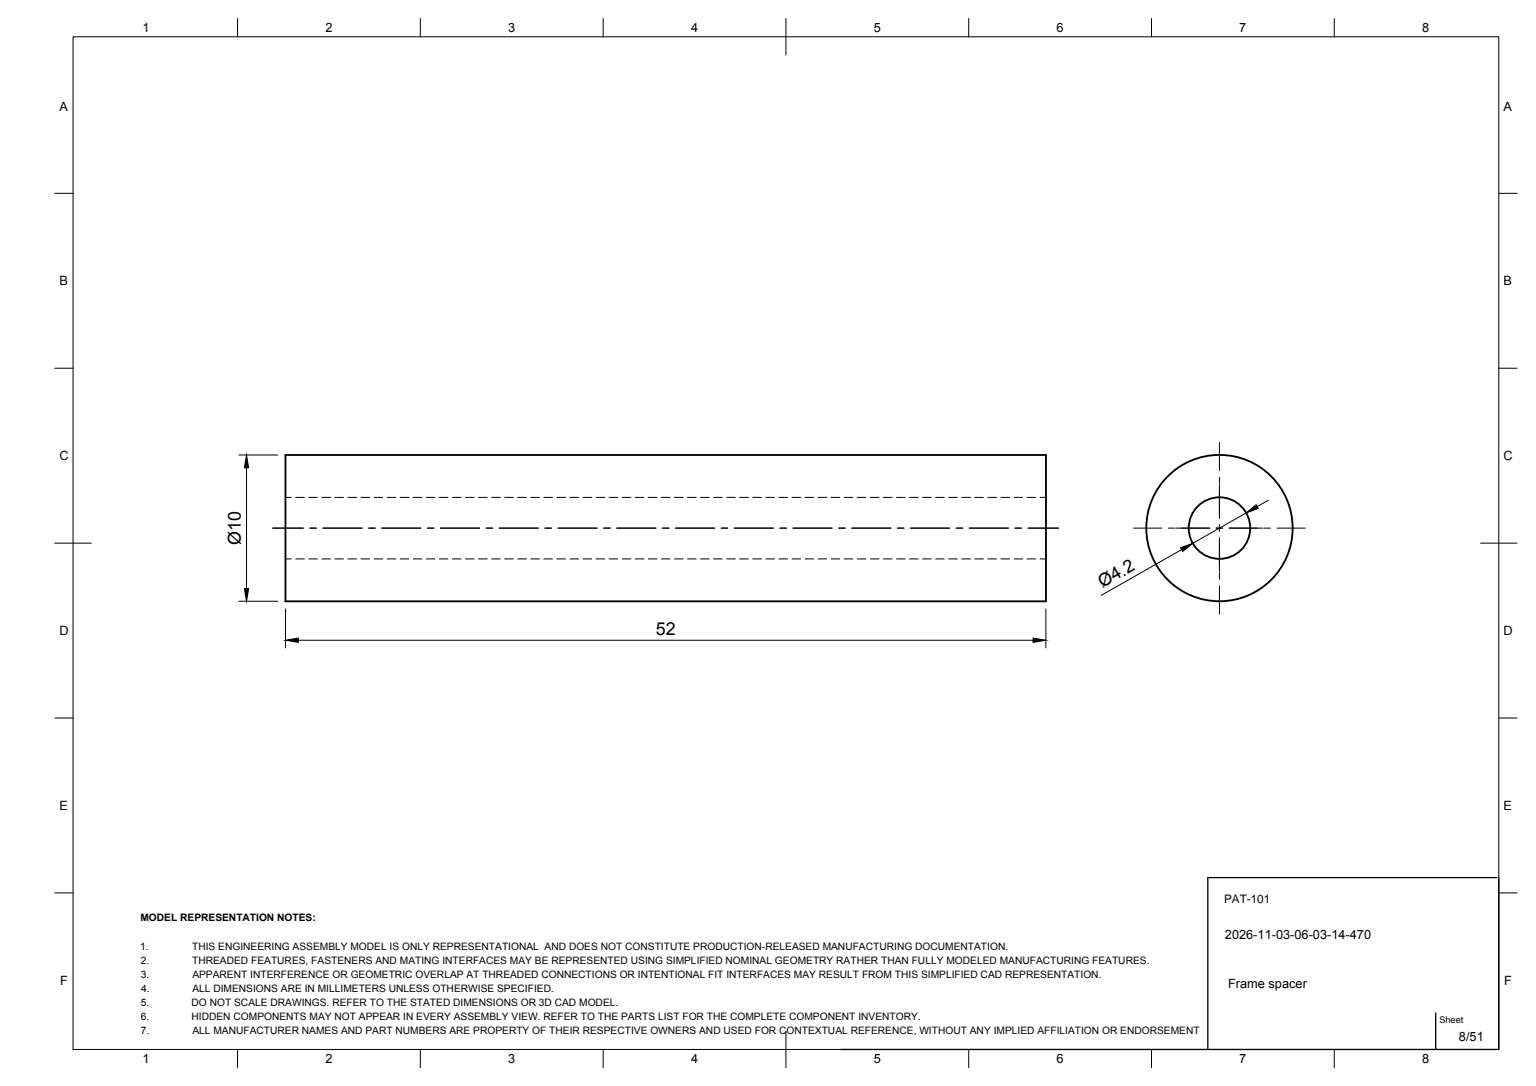
ISO-10303-21;
HEADER;
/* Generated by software containing ST-Developer
 * from STEP Tools, Inc. (www.steptools.com) 
 */

FILE_DESCRIPTION(
/* description */ ('Spur gear reduction stage 2-1 on bearing plates'),
/* implementation_level */ '2;1');

FILE_NAME(
/* name */ 'Frame spacer.step',
/* time_stamp */ '2026-10-28T03:22:07-07:00',
/* author */ (''),
/* organization */ (''),
/* preprocessor_version */ 'ST-DEVELOPER v20.2',
/* originating_system */ 'Autodesk Translation Framework v15.17.0.0',
/* authorisation */ '');

FILE_SCHEMA (('AUTOMOTIVE_DESIGN { 1 0 10303 214 3 1 1 }'));
ENDSEC;

DATA;
#10=MECHANICAL_DESIGN_GEOMETRIC_PRESENTATION_REPRESENTATION('',(#950),#53909);
#864=SHAPE_REPRESENTATION_RELATIONSHIP('SRR','None',#54091,#907);
#907=ADVANCED_BREP_SHAPE_REPRESENTATION('',(#1008),#53865);
#950=STYLED_ITEM('',(#54376),#1008);
#1008=MANIFOLD_SOLID_BREP('Body1',#11274);
#1132=FACE_BOUND('',#2304,.T.);
#1133=FACE_BOUND('',#2306,.T.);
#1272=PLANE('',#11984);
#1273=PLANE('',#11985);
#1581=FACE_OUTER_BOUND('',#2301,.T.);
#1582=FACE_OUTER_BOUND('',#2302,.T.);
#1583=FACE_OUTER_BOUND('',#2303,.T.);
#1584=FACE_OUTER_BOUND('',#2305,.T.);
#2301=EDGE_LOOP('',(#7688,#7689,#7690,#7691));
#2302=EDGE_LOOP('',(#7692,#7693,#7694,#7695));
#2303=EDGE_LOOP('',(#7696));
#2304=EDGE_LOOP('',(#7697));
#2305=EDGE_LOOP('',(#7698));
#2306=EDGE_LOOP('',(#7699));
#3057=LINE('',#16343,#3698);
#3058=LINE('',#16349,#3699);
#3698=VECTOR('',#13410,0.21);
#3699=VECTOR('',#13417,0.5);
#4347=CIRCLE('',#11979,0.21);
#4348=CIRCLE('',#11980,0.21);
#4349=CIRCLE('',#11982,0.5);
#4350=CIRCLE('',#11983,0.5);
#4896=VERTEX_POINT('',#16340);
#4897=VERTEX_POINT('',#16342);
#4898=VERTEX_POINT('',#16346);
#4899=VERTEX_POINT('',#16348);
#5986=EDGE_CURVE('',#4896,#4896,#4347,.T.);
#5987=EDGE_CURVE('',#4896,#4897,#3057,.T.);
#5988=EDGE_CURVE('',#4897,#4897,#4348,.T.);
#5989=EDGE_CURVE('',#4898,#4898,#4349,.T.);
#5990=EDGE_CURVE('',#4898,#4899,#3058,.T.);
#5991=EDGE_CURVE('',#4899,#4899,#4350,.T.);
#7688=ORIENTED_EDGE('',*,*,#5986,.F.);
#7689=ORIENTED_EDGE('',*,*,#5987,.T.);
#7690=ORIENTED_EDGE('',*,*,#5988,.T.);
#7691=ORIENTED_EDGE('',*,*,#5987,.F.);
#7692=ORIENTED_EDGE('',*,*,#5989,.F.);
#7693=ORIENTED_EDGE('',*,*,#5990,.T.);
#7694=ORIENTED_EDGE('',*,*,#5991,.T.);
#7695=ORIENTED_EDGE('',*,*,#5990,.F.);
#7696=ORIENTED_EDGE('',*,*,#5989,.T.);
#7697=ORIENTED_EDGE('',*,*,#5986,.T.);
#7698=ORIENTED_EDGE('',*,*,#5991,.F.);
#7699=ORIENTED_EDGE('',*,*,#5988,.F.);
#10464=CYLINDRICAL_SURFACE('',#11978,0.21);
#10465=CYLINDRICAL_SURFACE('',#11981,0.5);
#10701=ADVANCED_FACE('',(#1581),#10464,.F.);
#10702=ADVANCED_FACE('',(#1582),#10465,.T.);
#10703=ADVANCED_FACE('',(#1583,#1132),#1272,.T.);
#10704=ADVANCED_FACE('',(#1584,#1133),#1273,.F.);
#11274=CLOSED_SHELL('',(#10701,#10702,#10703,#10704));
#11977=AXIS2_PLACEMENT_3D('',#16338,#13404,#13405);
#11978=AXIS2_PLACEMENT_3D('',#16339,#13406,#13407);
#11979=AXIS2_PLACEMENT_3D('',#16341,#13408,#13409);
#11980=AXIS2_PLACEMENT_3D('',#16344,#13411,#13412);
#11981=AXIS2_PLACEMENT_3D('',#16345,#13413,#13414);
#11982=AXIS2_PLACEMENT_3D('',#16347,#13415,#13416);
#11983=AXIS2_PLACEMENT_3D('',#16350,#13418,#13419);
#11984=AXIS2_PLACEMENT_3D('',#16351,#13420,#13421);
#11985=AXIS2_PLACEMENT_3D('',#16352,#13422,#13423);
#13404=DIRECTION('axis',(0.,0.,1.));
#13405=DIRECTION('refdir',(1.,0.,0.));
#13406=DIRECTION('center_axis',(0.,1.,0.));
#13407=DIRECTION('ref_axis',(1.,0.,0.));
#13408=DIRECTION('center_axis',(0.,-1.,0.));
#13409=DIRECTION('ref_axis',(1.,0.,0.));
#13410=DIRECTION('',(0.,-1.,0.));
#13411=DIRECTION('center_axis',(0.,-1.,0.));
#13412=DIRECTION('ref_axis',(1.,0.,0.));
#13413=DIRECTION('center_axis',(0.,1.,0.));
#13414=DIRECTION('ref_axis',(1.,0.,0.));
#13415=DIRECTION('center_axis',(0.,1.,0.));
#13416=DIRECTION('ref_axis',(1.,0.,0.));
#13417=DIRECTION('',(0.,-1.,0.));
#13418=DIRECTION('center_axis',(0.,1.,0.));
#13419=DIRECTION('ref_axis',(1.,0.,0.));
#13420=DIRECTION('center_axis',(0.,1.,0.));
#13421=DIRECTION('ref_axis',(1.,0.,0.));
#13422=DIRECTION('center_axis',(0.,1.,0.));
#13423=DIRECTION('ref_axis',(1.,0.,0.));
#16338=CARTESIAN_POINT('',(0.,0.,0.));
#16339=CARTESIAN_POINT('Origin',(-2.,-2.6,2.));
#16340=CARTESIAN_POINT('',(-2.21,2.6,2.));
#16341=CARTESIAN_POINT('Origin',(-2.,2.6,2.));
#16342=CARTESIAN_POINT('',(-2.21,-2.6,2.));
#16343=CARTESIAN_POINT('',(-2.21,-2.6,2.));
#16344=CARTESIAN_POINT('Origin',(-2.,-2.6,2.));
#16345=CARTESIAN_POINT('Origin',(-2.,-2.6,2.));
#16346=CARTESIAN_POINT('',(-2.5,2.6,2.));
#16347=CARTESIAN_POINT('Origin',(-2.,2.6,2.));
#16348=CARTESIAN_POINT('',(-2.5,-2.6,2.));
#16349=CARTESIAN_POINT('',(-2.5,-2.6,2.));
#16350=CARTESIAN_POINT('Origin',(-2.,-2.6,2.));
#16351=CARTESIAN_POINT('Origin',(-2.,2.6,2.));
#16352=CARTESIAN_POINT('Origin',(-2.,-2.6,2.));
#53815=UNCERTAINTY_MEASURE_WITH_UNIT(LENGTH_MEASURE(0.001),#53910,
'DISTANCE_ACCURACY_VALUE',
'Maximum model space distance between geometric entities at asserted c
onnectivities');
#53859=UNCERTAINTY_MEASURE_WITH_UNIT(LENGTH_MEASURE(0.001),#53910,
'DISTANCE_ACCURACY_VALUE',
'Maximum model space distance between geometric entities at asserted c
onnectivities');
#53865=(
GEOMETRIC_REPRESENTATION_CONTEXT(3)
GLOBAL_UNCERTAINTY_ASSIGNED_CONTEXT((#53815))
GLOBAL_UNIT_ASSIGNED_CONTEXT((#53910,#53912,#53913))
REPRESENTATION_CONTEXT('','3D')
);
#53909=(
GEOMETRIC_REPRESENTATION_CONTEXT(3)
GLOBAL_UNCERTAINTY_ASSIGNED_CONTEXT((#53859))
GLOBAL_UNIT_ASSIGNED_CONTEXT((#53910,#53912,#53913))
REPRESENTATION_CONTEXT('','3D')
);
#53910=(
LENGTH_UNIT()
NAMED_UNIT(*)
SI_UNIT(.CENTI.,.METRE.)
);
#53912=(
NAMED_UNIT(*)
PLANE_ANGLE_UNIT()
SI_UNIT($,.RADIAN.)
);
#53913=(
NAMED_UNIT(*)
SI_UNIT($,.STERADIAN.)
SOLID_ANGLE_UNIT()
);
#53919=SHAPE_DEFINITION_REPRESENTATION(#53968,#54091);
#53968=PRODUCT_DEFINITION_SHAPE('',$,#54141);
#54091=SHAPE_REPRESENTATION('',(#11977),#53865);
#54135=PRODUCT_DEFINITION_CONTEXT('part definition',#54284,'design');
#54141=PRODUCT_DEFINITION('Frame spacer','Frame spacer',#54190,#54135);
#54190=PRODUCT_DEFINITION_FORMATION('',$,#54291);
#54284=APPLICATION_CONTEXT(
'Core Data for Automotive Mechanical Design Process');
#54285=PRODUCT_CONTEXT('part definition',#54284,'mechanical');
#54291=PRODUCT('Frame spacer','Frame spacer','Frame spacer',(#54285));
#54370=COLOUR_RGB('Dark Blue',0.08,0.2,0.34);
#54371=FILL_AREA_STYLE_COLOUR('',#54370);
#54372=FILL_AREA_STYLE('',(#54371));
#54373=SURFACE_STYLE_FILL_AREA(#54372);
#54374=SURFACE_SIDE_STYLE('',(#54373));
#54375=SURFACE_STYLE_USAGE(.BOTH.,#54374);
#54376=PRESENTATION_STYLE_ASSIGNMENT((#54375));
ENDSEC;
END-ISO-10303-21;
